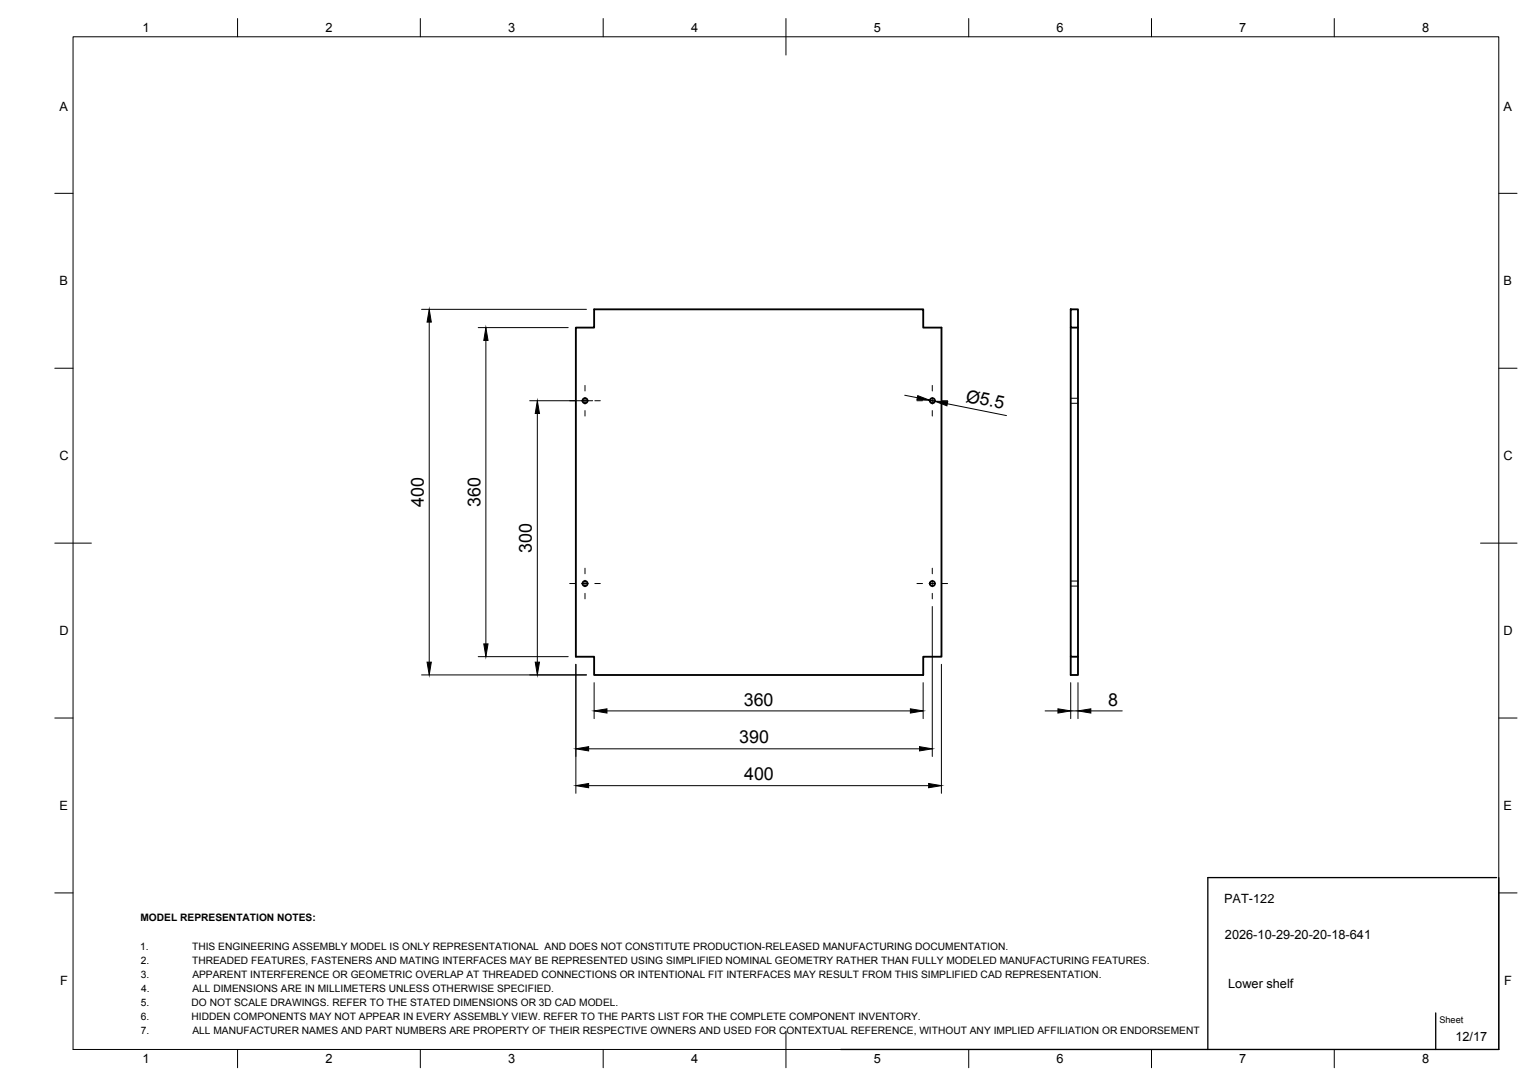
ISO-10303-21;
HEADER;
/* Generated by software containing ST-Developer
 * from STEP Tools, Inc. (www.steptools.com) 
 */

FILE_DESCRIPTION(
/* description */ ('PAT-122'),
/* implementation_level */ '2;1');

FILE_NAME(
/* name */ 'Lower shelf.step',
/* time_stamp */ '2026-10-29T20:20:12-07:00',
/* author */ (''),
/* organization */ (''),
/* preprocessor_version */ 'ST-DEVELOPER v20.2',
/* originating_system */ 'Autodesk Translation Framework v15.17.0.0',
/* authorisation */ '');

FILE_SCHEMA (('AUTOMOTIVE_DESIGN { 1 0 10303 214 3 1 1 }'));
ENDSEC;

DATA;
#10=MECHANICAL_DESIGN_GEOMETRIC_PRESENTATION_REPRESENTATION('',(#500),#10019);
#456=SHAPE_REPRESENTATION_RELATIONSHIP('SRR','None',#10177,#478);
#478=ADVANCED_BREP_SHAPE_REPRESENTATION('',(#522),#10006);
#500=STYLED_ITEM('',(#10341),#522);
#522=MANIFOLD_SOLID_BREP('Body1',#5622);
#559=FACE_BOUND('',#1203,.T.);
#560=FACE_BOUND('',#1204,.T.);
#561=FACE_BOUND('',#1205,.T.);
#562=FACE_BOUND('',#1206,.T.);
#563=FACE_BOUND('',#1217,.T.);
#564=FACE_BOUND('',#1218,.T.);
#565=FACE_BOUND('',#1219,.T.);
#566=FACE_BOUND('',#1220,.T.);
#635=PLANE('',#6003);
#636=PLANE('',#6004);
#637=PLANE('',#6005);
#638=PLANE('',#6006);
#639=PLANE('',#6007);
#640=PLANE('',#6008);
#641=PLANE('',#6009);
#642=PLANE('',#6010);
#643=PLANE('',#6011);
#644=PLANE('',#6012);
#645=PLANE('',#6013);
#646=PLANE('',#6014);
#647=PLANE('',#6015);
#648=PLANE('',#6016);
#875=FACE_OUTER_BOUND('',#1195,.T.);
#876=FACE_OUTER_BOUND('',#1196,.T.);
#877=FACE_OUTER_BOUND('',#1197,.T.);
#878=FACE_OUTER_BOUND('',#1198,.T.);
#879=FACE_OUTER_BOUND('',#1199,.T.);
#880=FACE_OUTER_BOUND('',#1200,.T.);
#881=FACE_OUTER_BOUND('',#1201,.T.);
#882=FACE_OUTER_BOUND('',#1202,.T.);
#883=FACE_OUTER_BOUND('',#1207,.T.);
#884=FACE_OUTER_BOUND('',#1208,.T.);
#885=FACE_OUTER_BOUND('',#1209,.T.);
#886=FACE_OUTER_BOUND('',#1210,.T.);
#887=FACE_OUTER_BOUND('',#1211,.T.);
#888=FACE_OUTER_BOUND('',#1212,.T.);
#889=FACE_OUTER_BOUND('',#1213,.T.);
#890=FACE_OUTER_BOUND('',#1214,.T.);
#891=FACE_OUTER_BOUND('',#1215,.T.);
#892=FACE_OUTER_BOUND('',#1216,.T.);
#1195=EDGE_LOOP('',(#4033,#4034,#4035,#4036));
#1196=EDGE_LOOP('',(#4037,#4038,#4039,#4040));
#1197=EDGE_LOOP('',(#4041,#4042,#4043,#4044));
#1198=EDGE_LOOP('',(#4045,#4046,#4047,#4048));
#1199=EDGE_LOOP('',(#4049,#4050,#4051,#4052));
#1200=EDGE_LOOP('',(#4053,#4054,#4055,#4056));
#1201=EDGE_LOOP('',(#4057,#4058,#4059,#4060));
#1202=EDGE_LOOP('',(#4061,#4062,#4063,#4064,#4065,#4066,#4067,#4068,#4069,
#4070,#4071,#4072));
#1203=EDGE_LOOP('',(#4073));
#1204=EDGE_LOOP('',(#4074));
#1205=EDGE_LOOP('',(#4075));
#1206=EDGE_LOOP('',(#4076));
#1207=EDGE_LOOP('',(#4077,#4078,#4079,#4080));
#1208=EDGE_LOOP('',(#4081,#4082,#4083,#4084));
#1209=EDGE_LOOP('',(#4085,#4086,#4087,#4088));
#1210=EDGE_LOOP('',(#4089,#4090,#4091,#4092));
#1211=EDGE_LOOP('',(#4093,#4094,#4095,#4096));
#1212=EDGE_LOOP('',(#4097,#4098,#4099,#4100));
#1213=EDGE_LOOP('',(#4101,#4102,#4103,#4104));
#1214=EDGE_LOOP('',(#4105,#4106,#4107,#4108));
#1215=EDGE_LOOP('',(#4109,#4110,#4111,#4112));
#1216=EDGE_LOOP('',(#4113,#4114,#4115,#4116,#4117,#4118,#4119,#4120,#4121,
#4122,#4123,#4124));
#1217=EDGE_LOOP('',(#4125));
#1218=EDGE_LOOP('',(#4126));
#1219=EDGE_LOOP('',(#4127));
#1220=EDGE_LOOP('',(#4128));
#1523=LINE('',#8263,#2067);
#1524=LINE('',#8269,#2068);
#1525=LINE('',#8275,#2069);
#1526=LINE('',#8281,#2070);
#1527=LINE('',#8286,#2071);
#1528=LINE('',#8288,#2072);
#1529=LINE('',#8290,#2073);
#1530=LINE('',#8291,#2074);
#1531=LINE('',#8294,#2075);
#1532=LINE('',#8296,#2076);
#1533=LINE('',#8297,#2077);
#1534=LINE('',#8300,#2078);
#1535=LINE('',#8302,#2079);
#1536=LINE('',#8303,#2080);
#1537=LINE('',#8306,#2081);
#1538=LINE('',#8308,#2082);
#1539=LINE('',#8310,#2083);
#1540=LINE('',#8312,#2084);
#1541=LINE('',#8314,#2085);
#1542=LINE('',#8316,#2086);
#1543=LINE('',#8318,#2087);
#1544=LINE('',#8320,#2088);
#1545=LINE('',#8321,#2089);
#1546=LINE('',#8325,#2090);
#1547=LINE('',#8326,#2091);
#1548=LINE('',#8327,#2092);
#1549=LINE('',#8329,#2093);
#1550=LINE('',#8332,#2094);
#1551=LINE('',#8333,#2095);
#1552=LINE('',#8337,#2096);
#1553=LINE('',#8338,#2097);
#1554=LINE('',#8339,#2098);
#1555=LINE('',#8342,#2099);
#1556=LINE('',#8343,#2100);
#1557=LINE('',#8345,#2101);
#1558=LINE('',#8348,#2102);
#1559=LINE('',#8349,#2103);
#1560=LINE('',#8352,#2104);
#1561=LINE('',#8353,#2105);
#1562=LINE('',#8355,#2106);
#2067=VECTOR('',#6684,0.274999999999999);
#2068=VECTOR('',#6691,0.274999999999999);
#2069=VECTOR('',#6698,0.274999999999999);
#2070=VECTOR('',#6705,0.274999999999999);
#2071=VECTOR('',#6710,1.);
#2072=VECTOR('',#6711,1.);
#2073=VECTOR('',#6712,1.);
#2074=VECTOR('',#6713,1.);
#2075=VECTOR('',#6716,1.);
#2076=VECTOR('',#6717,1.);
#2077=VECTOR('',#6718,1.);
#2078=VECTOR('',#6721,1.);
#2079=VECTOR('',#6722,1.);
#2080=VECTOR('',#6723,1.);
#2081=VECTOR('',#6726,1.);
#2082=VECTOR('',#6727,1.);
#2083=VECTOR('',#6728,1.);
#2084=VECTOR('',#6729,1.);
#2085=VECTOR('',#6730,1.);
#2086=VECTOR('',#6731,1.);
#2087=VECTOR('',#6732,1.);
#2088=VECTOR('',#6733,1.);
#2089=VECTOR('',#6734,1.);
#2090=VECTOR('',#6737,1.);
#2091=VECTOR('',#6738,1.);
#2092=VECTOR('',#6739,1.);
#2093=VECTOR('',#6742,1.);
#2094=VECTOR('',#6745,1.);
#2095=VECTOR('',#6746,1.);
#2096=VECTOR('',#6749,1.);
#2097=VECTOR('',#6750,1.);
#2098=VECTOR('',#6751,1.);
#2099=VECTOR('',#6754,1.);
#2100=VECTOR('',#6755,1.);
#2101=VECTOR('',#6758,1.);
#2102=VECTOR('',#6761,1.);
#2103=VECTOR('',#6762,1.);
#2104=VECTOR('',#6765,1.);
#2105=VECTOR('',#6766,1.);
#2106=VECTOR('',#6769,1.);
#2623=CIRCLE('',#5992,0.274999999999999);
#2624=CIRCLE('',#5993,0.274999999999999);
#2625=CIRCLE('',#5995,0.274999999999999);
#2626=CIRCLE('',#5996,0.274999999999999);
#2627=CIRCLE('',#5998,0.274999999999999);
#2628=CIRCLE('',#5999,0.274999999999999);
#2629=CIRCLE('',#6001,0.274999999999999);
#2630=CIRCLE('',#6002,0.274999999999999);
#2761=VERTEX_POINT('',#8260);
#2762=VERTEX_POINT('',#8262);
#2763=VERTEX_POINT('',#8266);
#2764=VERTEX_POINT('',#8268);
#2765=VERTEX_POINT('',#8272);
#2766=VERTEX_POINT('',#8274);
#2767=VERTEX_POINT('',#8278);
#2768=VERTEX_POINT('',#8280);
#2769=VERTEX_POINT('',#8284);
#2770=VERTEX_POINT('',#8285);
#2771=VERTEX_POINT('',#8287);
#2772=VERTEX_POINT('',#8289);
#2773=VERTEX_POINT('',#8293);
#2774=VERTEX_POINT('',#8295);
#2775=VERTEX_POINT('',#8299);
#2776=VERTEX_POINT('',#8301);
#2777=VERTEX_POINT('',#8305);
#2778=VERTEX_POINT('',#8307);
#2779=VERTEX_POINT('',#8309);
#2780=VERTEX_POINT('',#8311);
#2781=VERTEX_POINT('',#8313);
#2782=VERTEX_POINT('',#8315);
#2783=VERTEX_POINT('',#8317);
#2784=VERTEX_POINT('',#8319);
#2785=VERTEX_POINT('',#8323);
#2786=VERTEX_POINT('',#8324);
#2787=VERTEX_POINT('',#8331);
#2788=VERTEX_POINT('',#8335);
#2789=VERTEX_POINT('',#8336);
#2790=VERTEX_POINT('',#8341);
#2791=VERTEX_POINT('',#8347);
#2792=VERTEX_POINT('',#8351);
#3251=EDGE_CURVE('',#2761,#2761,#2623,.T.);
#3252=EDGE_CURVE('',#2761,#2762,#1523,.T.);
#3253=EDGE_CURVE('',#2762,#2762,#2624,.T.);
#3254=EDGE_CURVE('',#2763,#2763,#2625,.T.);
#3255=EDGE_CURVE('',#2763,#2764,#1524,.T.);
#3256=EDGE_CURVE('',#2764,#2764,#2626,.T.);
#3257=EDGE_CURVE('',#2765,#2765,#2627,.T.);
#3258=EDGE_CURVE('',#2765,#2766,#1525,.T.);
#3259=EDGE_CURVE('',#2766,#2766,#2628,.T.);
#3260=EDGE_CURVE('',#2767,#2767,#2629,.T.);
#3261=EDGE_CURVE('',#2767,#2768,#1526,.T.);
#3262=EDGE_CURVE('',#2768,#2768,#2630,.T.);
#3263=EDGE_CURVE('',#2769,#2770,#1527,.T.);
#3264=EDGE_CURVE('',#2769,#2771,#1528,.T.);
#3265=EDGE_CURVE('',#2772,#2771,#1529,.T.);
#3266=EDGE_CURVE('',#2770,#2772,#1530,.T.);
#3267=EDGE_CURVE('',#2773,#2769,#1531,.T.);
#3268=EDGE_CURVE('',#2774,#2773,#1532,.T.);
#3269=EDGE_CURVE('',#2771,#2774,#1533,.T.);
#3270=EDGE_CURVE('',#2775,#2772,#1534,.T.);
#3271=EDGE_CURVE('',#2775,#2776,#1535,.T.);
#3272=EDGE_CURVE('',#2776,#2770,#1536,.T.);
#3273=EDGE_CURVE('',#2774,#2777,#1537,.T.);
#3274=EDGE_CURVE('',#2777,#2778,#1538,.T.);
#3275=EDGE_CURVE('',#2778,#2779,#1539,.T.);
#3276=EDGE_CURVE('',#2779,#2780,#1540,.T.);
#3277=EDGE_CURVE('',#2780,#2781,#1541,.T.);
#3278=EDGE_CURVE('',#2781,#2782,#1542,.T.);
#3279=EDGE_CURVE('',#2782,#2783,#1543,.T.);
#3280=EDGE_CURVE('',#2783,#2784,#1544,.T.);
#3281=EDGE_CURVE('',#2784,#2775,#1545,.T.);
#3282=EDGE_CURVE('',#2785,#2786,#1546,.T.);
#3283=EDGE_CURVE('',#2785,#2784,#1547,.T.);
#3284=EDGE_CURVE('',#2786,#2783,#1548,.T.);
#3285=EDGE_CURVE('',#2776,#2785,#1549,.T.);
#3286=EDGE_CURVE('',#2782,#2787,#1550,.T.);
#3287=EDGE_CURVE('',#2787,#2786,#1551,.T.);
#3288=EDGE_CURVE('',#2788,#2789,#1552,.T.);
#3289=EDGE_CURVE('',#2788,#2778,#1553,.T.);
#3290=EDGE_CURVE('',#2789,#2777,#1554,.T.);
#3291=EDGE_CURVE('',#2790,#2788,#1555,.T.);
#3292=EDGE_CURVE('',#2779,#2790,#1556,.T.);
#3293=EDGE_CURVE('',#2773,#2789,#1557,.T.);
#3294=EDGE_CURVE('',#2791,#2781,#1558,.T.);
#3295=EDGE_CURVE('',#2787,#2791,#1559,.T.);
#3296=EDGE_CURVE('',#2792,#2780,#1560,.T.);
#3297=EDGE_CURVE('',#2791,#2792,#1561,.T.);
#3298=EDGE_CURVE('',#2790,#2792,#1562,.T.);
#4033=ORIENTED_EDGE('',*,*,#3251,.F.);
#4034=ORIENTED_EDGE('',*,*,#3252,.T.);
#4035=ORIENTED_EDGE('',*,*,#3253,.F.);
#4036=ORIENTED_EDGE('',*,*,#3252,.F.);
#4037=ORIENTED_EDGE('',*,*,#3254,.F.);
#4038=ORIENTED_EDGE('',*,*,#3255,.T.);
#4039=ORIENTED_EDGE('',*,*,#3256,.F.);
#4040=ORIENTED_EDGE('',*,*,#3255,.F.);
#4041=ORIENTED_EDGE('',*,*,#3257,.F.);
#4042=ORIENTED_EDGE('',*,*,#3258,.T.);
#4043=ORIENTED_EDGE('',*,*,#3259,.F.);
#4044=ORIENTED_EDGE('',*,*,#3258,.F.);
#4045=ORIENTED_EDGE('',*,*,#3260,.F.);
#4046=ORIENTED_EDGE('',*,*,#3261,.T.);
#4047=ORIENTED_EDGE('',*,*,#3262,.F.);
#4048=ORIENTED_EDGE('',*,*,#3261,.F.);
#4049=ORIENTED_EDGE('',*,*,#3263,.F.);
#4050=ORIENTED_EDGE('',*,*,#3264,.T.);
#4051=ORIENTED_EDGE('',*,*,#3265,.F.);
#4052=ORIENTED_EDGE('',*,*,#3266,.F.);
#4053=ORIENTED_EDGE('',*,*,#3267,.F.);
#4054=ORIENTED_EDGE('',*,*,#3268,.F.);
#4055=ORIENTED_EDGE('',*,*,#3269,.F.);
#4056=ORIENTED_EDGE('',*,*,#3264,.F.);
#4057=ORIENTED_EDGE('',*,*,#3266,.T.);
#4058=ORIENTED_EDGE('',*,*,#3270,.F.);
#4059=ORIENTED_EDGE('',*,*,#3271,.T.);
#4060=ORIENTED_EDGE('',*,*,#3272,.T.);
#4061=ORIENTED_EDGE('',*,*,#3265,.T.);
#4062=ORIENTED_EDGE('',*,*,#3269,.T.);
#4063=ORIENTED_EDGE('',*,*,#3273,.T.);
#4064=ORIENTED_EDGE('',*,*,#3274,.T.);
#4065=ORIENTED_EDGE('',*,*,#3275,.T.);
#4066=ORIENTED_EDGE('',*,*,#3276,.T.);
#4067=ORIENTED_EDGE('',*,*,#3277,.T.);
#4068=ORIENTED_EDGE('',*,*,#3278,.T.);
#4069=ORIENTED_EDGE('',*,*,#3279,.T.);
#4070=ORIENTED_EDGE('',*,*,#3280,.T.);
#4071=ORIENTED_EDGE('',*,*,#3281,.T.);
#4072=ORIENTED_EDGE('',*,*,#3270,.T.);
#4073=ORIENTED_EDGE('',*,*,#3253,.T.);
#4074=ORIENTED_EDGE('',*,*,#3256,.T.);
#4075=ORIENTED_EDGE('',*,*,#3259,.T.);
#4076=ORIENTED_EDGE('',*,*,#3262,.T.);
#4077=ORIENTED_EDGE('',*,*,#3282,.F.);
#4078=ORIENTED_EDGE('',*,*,#3283,.T.);
#4079=ORIENTED_EDGE('',*,*,#3280,.F.);
#4080=ORIENTED_EDGE('',*,*,#3284,.F.);
#4081=ORIENTED_EDGE('',*,*,#3285,.F.);
#4082=ORIENTED_EDGE('',*,*,#3271,.F.);
#4083=ORIENTED_EDGE('',*,*,#3281,.F.);
#4084=ORIENTED_EDGE('',*,*,#3283,.F.);
#4085=ORIENTED_EDGE('',*,*,#3284,.T.);
#4086=ORIENTED_EDGE('',*,*,#3279,.F.);
#4087=ORIENTED_EDGE('',*,*,#3286,.T.);
#4088=ORIENTED_EDGE('',*,*,#3287,.T.);
#4089=ORIENTED_EDGE('',*,*,#3288,.F.);
#4090=ORIENTED_EDGE('',*,*,#3289,.T.);
#4091=ORIENTED_EDGE('',*,*,#3274,.F.);
#4092=ORIENTED_EDGE('',*,*,#3290,.F.);
#4093=ORIENTED_EDGE('',*,*,#3291,.F.);
#4094=ORIENTED_EDGE('',*,*,#3292,.F.);
#4095=ORIENTED_EDGE('',*,*,#3275,.F.);
#4096=ORIENTED_EDGE('',*,*,#3289,.F.);
#4097=ORIENTED_EDGE('',*,*,#3268,.T.);
#4098=ORIENTED_EDGE('',*,*,#3293,.T.);
#4099=ORIENTED_EDGE('',*,*,#3290,.T.);
#4100=ORIENTED_EDGE('',*,*,#3273,.F.);
#4101=ORIENTED_EDGE('',*,*,#3278,.F.);
#4102=ORIENTED_EDGE('',*,*,#3294,.F.);
#4103=ORIENTED_EDGE('',*,*,#3295,.F.);
#4104=ORIENTED_EDGE('',*,*,#3286,.F.);
#4105=ORIENTED_EDGE('',*,*,#3277,.F.);
#4106=ORIENTED_EDGE('',*,*,#3296,.F.);
#4107=ORIENTED_EDGE('',*,*,#3297,.F.);
#4108=ORIENTED_EDGE('',*,*,#3294,.T.);
#4109=ORIENTED_EDGE('',*,*,#3292,.T.);
#4110=ORIENTED_EDGE('',*,*,#3298,.T.);
#4111=ORIENTED_EDGE('',*,*,#3296,.T.);
#4112=ORIENTED_EDGE('',*,*,#3276,.F.);
#4113=ORIENTED_EDGE('',*,*,#3263,.T.);
#4114=ORIENTED_EDGE('',*,*,#3272,.F.);
#4115=ORIENTED_EDGE('',*,*,#3285,.T.);
#4116=ORIENTED_EDGE('',*,*,#3282,.T.);
#4117=ORIENTED_EDGE('',*,*,#3287,.F.);
#4118=ORIENTED_EDGE('',*,*,#3295,.T.);
#4119=ORIENTED_EDGE('',*,*,#3297,.T.);
#4120=ORIENTED_EDGE('',*,*,#3298,.F.);
#4121=ORIENTED_EDGE('',*,*,#3291,.T.);
#4122=ORIENTED_EDGE('',*,*,#3288,.T.);
#4123=ORIENTED_EDGE('',*,*,#3293,.F.);
#4124=ORIENTED_EDGE('',*,*,#3267,.T.);
#4125=ORIENTED_EDGE('',*,*,#3251,.T.);
#4126=ORIENTED_EDGE('',*,*,#3254,.T.);
#4127=ORIENTED_EDGE('',*,*,#3257,.T.);
#4128=ORIENTED_EDGE('',*,*,#3260,.T.);
#5285=CYLINDRICAL_SURFACE('',#5991,0.274999999999999);
#5286=CYLINDRICAL_SURFACE('',#5994,0.274999999999999);
#5287=CYLINDRICAL_SURFACE('',#5997,0.274999999999999);
#5288=CYLINDRICAL_SURFACE('',#6000,0.274999999999999);
#5371=ADVANCED_FACE('',(#875),#5285,.F.);
#5372=ADVANCED_FACE('',(#876),#5286,.F.);
#5373=ADVANCED_FACE('',(#877),#5287,.F.);
#5374=ADVANCED_FACE('',(#878),#5288,.F.);
#5375=ADVANCED_FACE('',(#879),#635,.F.);
#5376=ADVANCED_FACE('',(#880),#636,.F.);
#5377=ADVANCED_FACE('',(#881),#637,.T.);
#5378=ADVANCED_FACE('',(#882,#559,#560,#561,#562),#638,.T.);
#5379=ADVANCED_FACE('',(#883),#639,.F.);
#5380=ADVANCED_FACE('',(#884),#640,.F.);
#5381=ADVANCED_FACE('',(#885),#641,.T.);
#5382=ADVANCED_FACE('',(#886),#642,.F.);
#5383=ADVANCED_FACE('',(#887),#643,.F.);
#5384=ADVANCED_FACE('',(#888),#644,.T.);
#5385=ADVANCED_FACE('',(#889),#645,.F.);
#5386=ADVANCED_FACE('',(#890),#646,.F.);
#5387=ADVANCED_FACE('',(#891),#647,.T.);
#5388=ADVANCED_FACE('',(#892,#563,#564,#565,#566),#648,.F.);
#5622=CLOSED_SHELL('',(#5371,#5372,#5373,#5374,#5375,#5376,#5377,#5378,
#5379,#5380,#5381,#5382,#5383,#5384,#5385,#5386,#5387,#5388));
#5990=AXIS2_PLACEMENT_3D('',#8258,#6678,#6679);
#5991=AXIS2_PLACEMENT_3D('',#8259,#6680,#6681);
#5992=AXIS2_PLACEMENT_3D('',#8261,#6682,#6683);
#5993=AXIS2_PLACEMENT_3D('',#8264,#6685,#6686);
#5994=AXIS2_PLACEMENT_3D('',#8265,#6687,#6688);
#5995=AXIS2_PLACEMENT_3D('',#8267,#6689,#6690);
#5996=AXIS2_PLACEMENT_3D('',#8270,#6692,#6693);
#5997=AXIS2_PLACEMENT_3D('',#8271,#6694,#6695);
#5998=AXIS2_PLACEMENT_3D('',#8273,#6696,#6697);
#5999=AXIS2_PLACEMENT_3D('',#8276,#6699,#6700);
#6000=AXIS2_PLACEMENT_3D('',#8277,#6701,#6702);
#6001=AXIS2_PLACEMENT_3D('',#8279,#6703,#6704);
#6002=AXIS2_PLACEMENT_3D('',#8282,#6706,#6707);
#6003=AXIS2_PLACEMENT_3D('',#8283,#6708,#6709);
#6004=AXIS2_PLACEMENT_3D('',#8292,#6714,#6715);
#6005=AXIS2_PLACEMENT_3D('',#8298,#6719,#6720);
#6006=AXIS2_PLACEMENT_3D('',#8304,#6724,#6725);
#6007=AXIS2_PLACEMENT_3D('',#8322,#6735,#6736);
#6008=AXIS2_PLACEMENT_3D('',#8328,#6740,#6741);
#6009=AXIS2_PLACEMENT_3D('',#8330,#6743,#6744);
#6010=AXIS2_PLACEMENT_3D('',#8334,#6747,#6748);
#6011=AXIS2_PLACEMENT_3D('',#8340,#6752,#6753);
#6012=AXIS2_PLACEMENT_3D('',#8344,#6756,#6757);
#6013=AXIS2_PLACEMENT_3D('',#8346,#6759,#6760);
#6014=AXIS2_PLACEMENT_3D('',#8350,#6763,#6764);
#6015=AXIS2_PLACEMENT_3D('',#8354,#6767,#6768);
#6016=AXIS2_PLACEMENT_3D('',#8356,#6770,#6771);
#6678=DIRECTION('axis',(0.,0.,1.));
#6679=DIRECTION('refdir',(1.,0.,0.));
#6680=DIRECTION('center_axis',(0.,0.,1.));
#6681=DIRECTION('ref_axis',(1.,0.,0.));
#6682=DIRECTION('center_axis',(0.,0.,1.));
#6683=DIRECTION('ref_axis',(1.,0.,0.));
#6684=DIRECTION('',(0.,0.,1.));
#6685=DIRECTION('center_axis',(0.,0.,-1.));
#6686=DIRECTION('ref_axis',(1.,0.,0.));
#6687=DIRECTION('center_axis',(0.,0.,1.));
#6688=DIRECTION('ref_axis',(1.,0.,0.));
#6689=DIRECTION('center_axis',(0.,0.,1.));
#6690=DIRECTION('ref_axis',(1.,0.,0.));
#6691=DIRECTION('',(0.,0.,1.));
#6692=DIRECTION('center_axis',(0.,0.,-1.));
#6693=DIRECTION('ref_axis',(1.,0.,0.));
#6694=DIRECTION('center_axis',(0.,0.,1.));
#6695=DIRECTION('ref_axis',(1.,0.,0.));
#6696=DIRECTION('center_axis',(0.,0.,1.));
#6697=DIRECTION('ref_axis',(1.,0.,0.));
#6698=DIRECTION('',(0.,0.,1.));
#6699=DIRECTION('center_axis',(0.,0.,-1.));
#6700=DIRECTION('ref_axis',(1.,0.,0.));
#6701=DIRECTION('center_axis',(0.,0.,1.));
#6702=DIRECTION('ref_axis',(1.,0.,0.));
#6703=DIRECTION('center_axis',(0.,0.,1.));
#6704=DIRECTION('ref_axis',(1.,0.,0.));
#6705=DIRECTION('',(0.,0.,1.));
#6706=DIRECTION('center_axis',(0.,0.,-1.));
#6707=DIRECTION('ref_axis',(1.,0.,0.));
#6708=DIRECTION('center_axis',(0.,-1.,0.));
#6709=DIRECTION('ref_axis',(1.,0.,0.));
#6710=DIRECTION('',(1.,0.,0.));
#6711=DIRECTION('',(0.,0.,1.));
#6712=DIRECTION('',(-1.,0.,0.));
#6713=DIRECTION('',(0.,0.,1.));
#6714=DIRECTION('center_axis',(-1.,0.,0.));
#6715=DIRECTION('ref_axis',(0.,-1.,0.));
#6716=DIRECTION('',(0.,-1.,0.));
#6717=DIRECTION('',(0.,0.,-1.));
#6718=DIRECTION('',(0.,1.,0.));
#6719=DIRECTION('center_axis',(1.,0.,0.));
#6720=DIRECTION('ref_axis',(0.,1.,0.));
#6721=DIRECTION('',(0.,1.,0.));
#6722=DIRECTION('',(0.,0.,-1.));
#6723=DIRECTION('',(0.,1.,0.));
#6724=DIRECTION('center_axis',(0.,0.,1.));
#6725=DIRECTION('ref_axis',(1.,0.,0.));
#6726=DIRECTION('',(-1.,0.,0.));
#6727=DIRECTION('',(0.,-1.,0.));
#6728=DIRECTION('',(-1.,0.,0.));
#6729=DIRECTION('',(0.,-1.,0.));
#6730=DIRECTION('',(1.,0.,0.));
#6731=DIRECTION('',(0.,-1.,0.));
#6732=DIRECTION('',(1.,0.,0.));
#6733=DIRECTION('',(0.,1.,0.));
#6734=DIRECTION('',(1.,0.,0.));
#6735=DIRECTION('center_axis',(-1.,0.,0.));
#6736=DIRECTION('ref_axis',(0.,-1.,0.));
#6737=DIRECTION('',(0.,-1.,0.));
#6738=DIRECTION('',(0.,0.,1.));
#6739=DIRECTION('',(0.,0.,1.));
#6740=DIRECTION('center_axis',(0.,1.,0.));
#6741=DIRECTION('ref_axis',(-1.,0.,0.));
#6742=DIRECTION('',(-1.,0.,0.));
#6743=DIRECTION('center_axis',(0.,-1.,0.));
#6744=DIRECTION('ref_axis',(1.,0.,0.));
#6745=DIRECTION('',(0.,0.,-1.));
#6746=DIRECTION('',(1.,0.,0.));
#6747=DIRECTION('center_axis',(1.,0.,0.));
#6748=DIRECTION('ref_axis',(0.,1.,0.));
#6749=DIRECTION('',(0.,1.,0.));
#6750=DIRECTION('',(0.,0.,1.));
#6751=DIRECTION('',(0.,0.,1.));
#6752=DIRECTION('center_axis',(0.,-1.,0.));
#6753=DIRECTION('ref_axis',(1.,0.,0.));
#6754=DIRECTION('',(1.,0.,0.));
#6755=DIRECTION('',(0.,0.,-1.));
#6756=DIRECTION('center_axis',(0.,1.,0.));
#6757=DIRECTION('ref_axis',(-1.,0.,0.));
#6758=DIRECTION('',(-1.,0.,0.));
#6759=DIRECTION('center_axis',(1.,0.,0.));
#6760=DIRECTION('ref_axis',(0.,1.,0.));
#6761=DIRECTION('',(0.,0.,1.));
#6762=DIRECTION('',(0.,1.,0.));
#6763=DIRECTION('center_axis',(0.,1.,0.));
#6764=DIRECTION('ref_axis',(-1.,0.,0.));
#6765=DIRECTION('',(0.,0.,1.));
#6766=DIRECTION('',(-1.,0.,0.));
#6767=DIRECTION('center_axis',(-1.,0.,0.));
#6768=DIRECTION('ref_axis',(0.,-1.,0.));
#6769=DIRECTION('',(0.,-1.,0.));
#6770=DIRECTION('center_axis',(0.,0.,1.));
#6771=DIRECTION('ref_axis',(1.,0.,0.));
#8258=CARTESIAN_POINT('',(0.,0.,0.));
#8259=CARTESIAN_POINT('Origin',(19.,-10.,4.9));
#8260=CARTESIAN_POINT('',(18.725,-10.,5.));
#8261=CARTESIAN_POINT('Origin',(19.,-10.,5.));
#8262=CARTESIAN_POINT('',(18.725,-10.,5.8));
#8263=CARTESIAN_POINT('',(18.725,-10.,4.9));
#8264=CARTESIAN_POINT('Origin',(19.,-10.,5.8));
#8265=CARTESIAN_POINT('Origin',(-19.,10.,4.9));
#8266=CARTESIAN_POINT('',(-19.275,10.,5.));
#8267=CARTESIAN_POINT('Origin',(-19.,10.,5.));
#8268=CARTESIAN_POINT('',(-19.275,10.,5.8));
#8269=CARTESIAN_POINT('',(-19.275,10.,4.9));
#8270=CARTESIAN_POINT('Origin',(-19.,10.,5.8));
#8271=CARTESIAN_POINT('Origin',(-19.,-10.,4.9));
#8272=CARTESIAN_POINT('',(-19.275,-10.,5.));
#8273=CARTESIAN_POINT('Origin',(-19.,-10.,5.));
#8274=CARTESIAN_POINT('',(-19.275,-10.,5.8));
#8275=CARTESIAN_POINT('',(-19.275,-10.,4.9));
#8276=CARTESIAN_POINT('Origin',(-19.,-10.,5.8));
#8277=CARTESIAN_POINT('Origin',(19.,10.,4.9));
#8278=CARTESIAN_POINT('',(18.725,10.,5.));
#8279=CARTESIAN_POINT('Origin',(19.,10.,5.));
#8280=CARTESIAN_POINT('',(18.725,10.,5.8));
#8281=CARTESIAN_POINT('',(18.725,10.,4.9));
#8282=CARTESIAN_POINT('Origin',(19.,10.,5.8));
#8283=CARTESIAN_POINT('Origin',(18.,18.,4.9));
#8284=CARTESIAN_POINT('',(18.,18.,5.));
#8285=CARTESIAN_POINT('',(20.,18.,5.));
#8286=CARTESIAN_POINT('',(9.,18.,5.));
#8287=CARTESIAN_POINT('',(18.,18.,5.8));
#8288=CARTESIAN_POINT('',(18.,18.,4.9));
#8289=CARTESIAN_POINT('',(20.,18.,5.8));
#8290=CARTESIAN_POINT('',(9.,18.,5.8));
#8291=CARTESIAN_POINT('',(20.,18.,4.95));
#8292=CARTESIAN_POINT('Origin',(18.,20.,4.9));
#8293=CARTESIAN_POINT('',(18.,20.,5.));
#8294=CARTESIAN_POINT('',(18.,10.,5.));
#8295=CARTESIAN_POINT('',(18.,20.,5.8));
#8296=CARTESIAN_POINT('',(18.,20.,4.95));
#8297=CARTESIAN_POINT('',(18.,10.,5.8));
#8298=CARTESIAN_POINT('Origin',(20.,-20.,5.));
#8299=CARTESIAN_POINT('',(20.,-18.,5.8));
#8300=CARTESIAN_POINT('',(20.,-20.,5.8));
#8301=CARTESIAN_POINT('',(20.,-18.,5.));
#8302=CARTESIAN_POINT('',(20.,-18.,4.95));
#8303=CARTESIAN_POINT('',(20.,-20.,5.));
#8304=CARTESIAN_POINT('Origin',(0.,0.,5.8));
#8305=CARTESIAN_POINT('',(-18.,20.,5.8));
#8306=CARTESIAN_POINT('',(20.,20.,5.8));
#8307=CARTESIAN_POINT('',(-18.,18.,5.8));
#8308=CARTESIAN_POINT('',(-18.,9.,5.8));
#8309=CARTESIAN_POINT('',(-20.,18.,5.8));
#8310=CARTESIAN_POINT('',(-10.,18.,5.8));
#8311=CARTESIAN_POINT('',(-20.,-18.,5.8));
#8312=CARTESIAN_POINT('',(-20.,20.,5.8));
#8313=CARTESIAN_POINT('',(-18.,-18.,5.8));
#8314=CARTESIAN_POINT('',(-9.,-18.,5.8));
#8315=CARTESIAN_POINT('',(-18.,-20.,5.8));
#8316=CARTESIAN_POINT('',(-18.,-10.,5.8));
#8317=CARTESIAN_POINT('',(18.,-20.,5.8));
#8318=CARTESIAN_POINT('',(-20.,-20.,5.8));
#8319=CARTESIAN_POINT('',(18.,-18.,5.8));
#8320=CARTESIAN_POINT('',(18.,-9.,5.8));
#8321=CARTESIAN_POINT('',(10.,-18.,5.8));
#8322=CARTESIAN_POINT('Origin',(18.,-18.,4.9));
#8323=CARTESIAN_POINT('',(18.,-18.,5.));
#8324=CARTESIAN_POINT('',(18.,-20.,5.));
#8325=CARTESIAN_POINT('',(18.,-9.,5.));
#8326=CARTESIAN_POINT('',(18.,-18.,4.9));
#8327=CARTESIAN_POINT('',(18.,-20.,4.95));
#8328=CARTESIAN_POINT('Origin',(20.,-18.,4.9));
#8329=CARTESIAN_POINT('',(10.,-18.,5.));
#8330=CARTESIAN_POINT('Origin',(-20.,-20.,5.));
#8331=CARTESIAN_POINT('',(-18.,-20.,5.));
#8332=CARTESIAN_POINT('',(-18.,-20.,4.95));
#8333=CARTESIAN_POINT('',(-20.,-20.,5.));
#8334=CARTESIAN_POINT('Origin',(-18.,18.,4.9));
#8335=CARTESIAN_POINT('',(-18.,18.,5.));
#8336=CARTESIAN_POINT('',(-18.,20.,5.));
#8337=CARTESIAN_POINT('',(-18.,9.,5.));
#8338=CARTESIAN_POINT('',(-18.,18.,4.9));
#8339=CARTESIAN_POINT('',(-18.,20.,4.95));
#8340=CARTESIAN_POINT('Origin',(-20.,18.,4.9));
#8341=CARTESIAN_POINT('',(-20.,18.,5.));
#8342=CARTESIAN_POINT('',(-10.,18.,5.));
#8343=CARTESIAN_POINT('',(-20.,18.,4.95));
#8344=CARTESIAN_POINT('Origin',(20.,20.,5.));
#8345=CARTESIAN_POINT('',(20.,20.,5.));
#8346=CARTESIAN_POINT('Origin',(-18.,-20.,4.9));
#8347=CARTESIAN_POINT('',(-18.,-18.,5.));
#8348=CARTESIAN_POINT('',(-18.,-18.,4.9));
#8349=CARTESIAN_POINT('',(-18.,-10.,5.));
#8350=CARTESIAN_POINT('Origin',(-18.,-18.,4.9));
#8351=CARTESIAN_POINT('',(-20.,-18.,5.));
#8352=CARTESIAN_POINT('',(-20.,-18.,4.95));
#8353=CARTESIAN_POINT('',(-9.,-18.,5.));
#8354=CARTESIAN_POINT('Origin',(-20.,20.,5.));
#8355=CARTESIAN_POINT('',(-20.,20.,5.));
#8356=CARTESIAN_POINT('Origin',(0.,0.,5.));
#9982=UNCERTAINTY_MEASURE_WITH_UNIT(LENGTH_MEASURE(0.001),#10020,
'DISTANCE_ACCURACY_VALUE',
'Maximum model space distance between geometric entities at asserted c
onnectivities');
#9995=UNCERTAINTY_MEASURE_WITH_UNIT(LENGTH_MEASURE(0.001),#10020,
'DISTANCE_ACCURACY_VALUE',
'Maximum model space distance between geometric entities at asserted c
onnectivities');
#10006=(
GEOMETRIC_REPRESENTATION_CONTEXT(3)
GLOBAL_UNCERTAINTY_ASSIGNED_CONTEXT((#9982))
GLOBAL_UNIT_ASSIGNED_CONTEXT((#10020,#10022,#10023))
REPRESENTATION_CONTEXT('','3D')
);
#10019=(
GEOMETRIC_REPRESENTATION_CONTEXT(3)
GLOBAL_UNCERTAINTY_ASSIGNED_CONTEXT((#9995))
GLOBAL_UNIT_ASSIGNED_CONTEXT((#10020,#10022,#10023))
REPRESENTATION_CONTEXT('','3D')
);
#10020=(
LENGTH_UNIT()
NAMED_UNIT(*)
SI_UNIT(.CENTI.,.METRE.)
);
#10022=(
NAMED_UNIT(*)
PLANE_ANGLE_UNIT()
SI_UNIT($,.RADIAN.)
);
#10023=(
NAMED_UNIT(*)
SI_UNIT($,.STERADIAN.)
SOLID_ANGLE_UNIT()
);
#10034=SHAPE_DEFINITION_REPRESENTATION(#10057,#10177);
#10057=PRODUCT_DEFINITION_SHAPE('',$,#10201);
#10177=SHAPE_REPRESENTATION('',(#5990),#10006);
#10190=PRODUCT_DEFINITION_CONTEXT('part definition',#10261,'design');
#10201=PRODUCT_DEFINITION('Lower shelf','Lower shelf',#10224,
#10190);
#10224=PRODUCT_DEFINITION_FORMATION('',$,#10273);
#10261=APPLICATION_CONTEXT(
'Core Data for Automotive Mechanical Design Process');
#10262=PRODUCT_CONTEXT('part definition',#10261,'mechanical');
#10273=PRODUCT('Lower shelf','Lower shelf','Lower shelf',(#10262));
#10335=COLOUR_RGB('Sky Blue',0.24,0.69,0.87);
#10336=FILL_AREA_STYLE_COLOUR('',#10335);
#10337=FILL_AREA_STYLE('',(#10336));
#10338=SURFACE_STYLE_FILL_AREA(#10337);
#10339=SURFACE_SIDE_STYLE('',(#10338));
#10340=SURFACE_STYLE_USAGE(.BOTH.,#10339);
#10341=PRESENTATION_STYLE_ASSIGNMENT((#10340));
ENDSEC;
END-ISO-10303-21;
